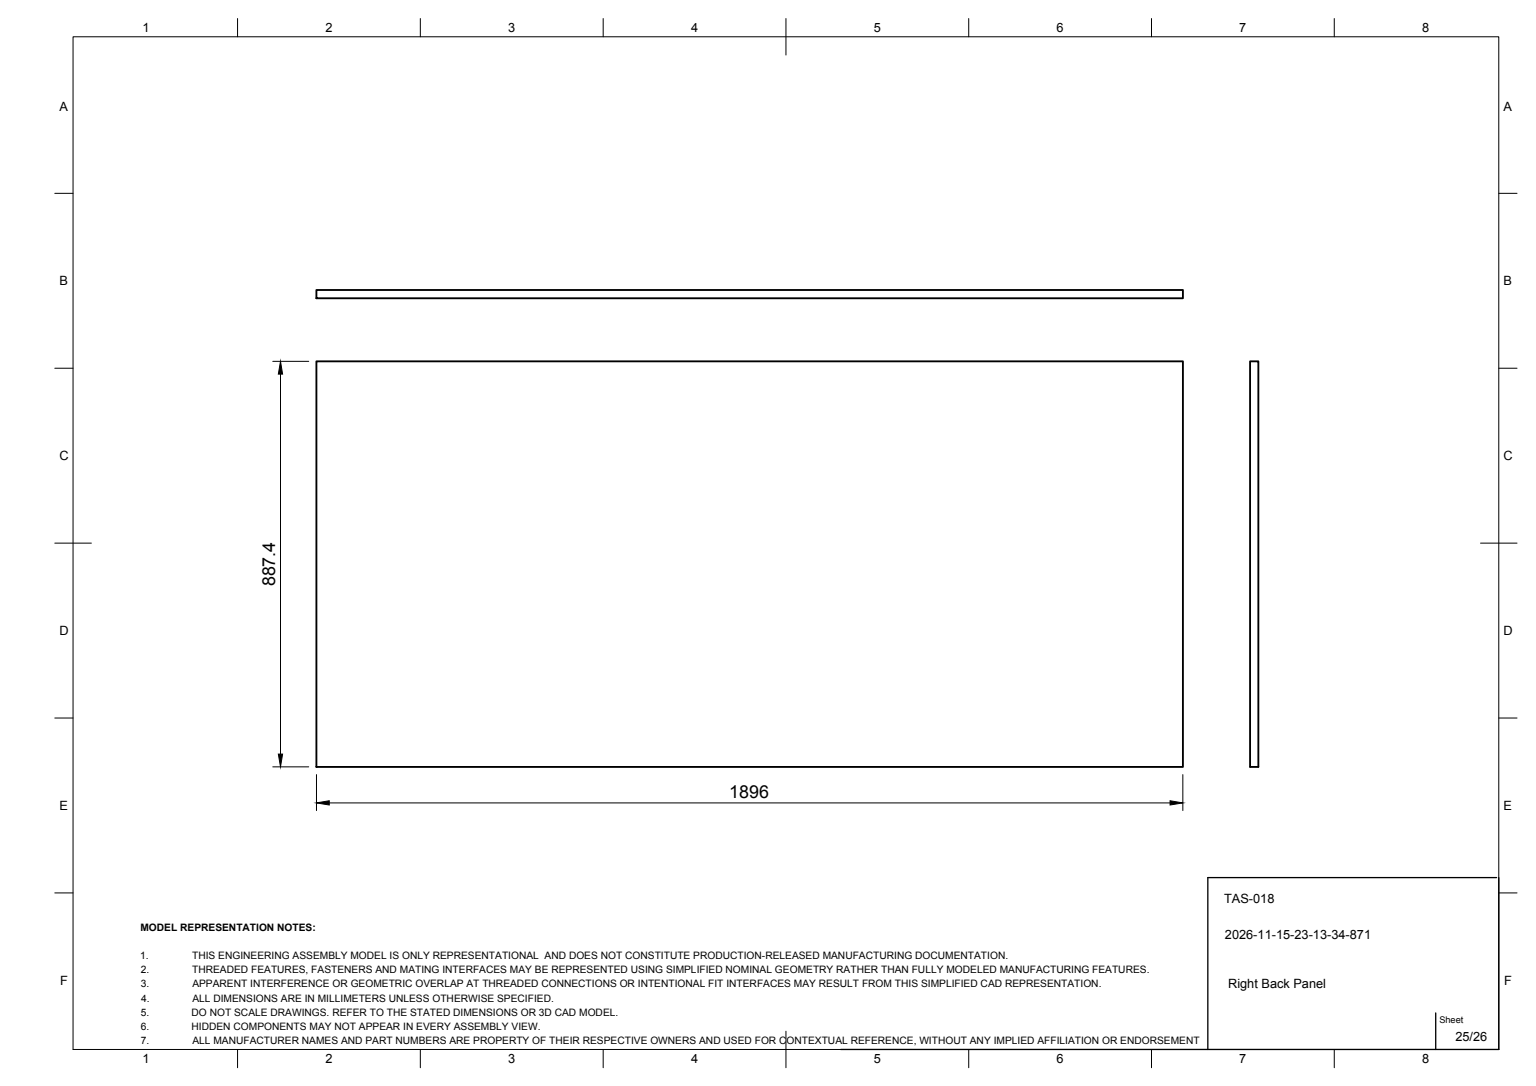
ISO-10303-21;
HEADER;
/* Generated by software containing ST-Developer
 * from STEP Tools, Inc. (www.steptools.com) 
 */

FILE_DESCRIPTION(
/* description */ (''),
/* implementation_level */ '2;1');

FILE_NAME(
/* name */ 'Right Back Panel.step',
/* time_stamp */ '2026-11-15T15:17:57-08:00',
/* author */ (''),
/* organization */ (''),
/* preprocessor_version */ 'ST-DEVELOPER v20.2',
/* originating_system */ 'Autodesk Translation Framework v15.17.0.0',
/* authorisation */ '');

FILE_SCHEMA (('AUTOMOTIVE_DESIGN { 1 0 10303 214 3 1 1 }'));
ENDSEC;

DATA;
#10=MECHANICAL_DESIGN_GEOMETRIC_PRESENTATION_REPRESENTATION('',(#200),#3723);
#152=SHAPE_REPRESENTATION_RELATIONSHIP('SRR','None',#3833,#176);
#176=ADVANCED_BREP_SHAPE_REPRESENTATION('',(#224),#3722);
#200=STYLED_ITEM('',(#3949),#224);
#224=MANIFOLD_SOLID_BREP('Body1',#2048);
#345=FACE_OUTER_BOUND('',#471,.T.);
#346=FACE_OUTER_BOUND('',#472,.T.);
#347=FACE_OUTER_BOUND('',#473,.T.);
#348=FACE_OUTER_BOUND('',#474,.T.);
#349=FACE_OUTER_BOUND('',#475,.T.);
#350=FACE_OUTER_BOUND('',#476,.T.);
#471=EDGE_LOOP('',(#1755,#1756,#1757,#1758));
#472=EDGE_LOOP('',(#1759,#1760,#1761,#1762));
#473=EDGE_LOOP('',(#1763,#1764,#1765,#1766));
#474=EDGE_LOOP('',(#1767,#1768,#1769,#1770));
#475=EDGE_LOOP('',(#1771,#1772,#1773,#1774));
#476=EDGE_LOOP('',(#1775,#1776,#1777,#1778));
#687=LINE('',#3623,#909);
#688=LINE('',#3625,#910);
#689=LINE('',#3627,#911);
#690=LINE('',#3628,#912);
#691=LINE('',#3631,#913);
#692=LINE('',#3633,#914);
#693=LINE('',#3634,#915);
#694=LINE('',#3637,#916);
#695=LINE('',#3639,#917);
#696=LINE('',#3640,#918);
#697=LINE('',#3642,#919);
#698=LINE('',#3643,#920);
#909=VECTOR('',#3033,74.6456692913386);
#910=VECTOR('',#3034,0.708661417322834);
#911=VECTOR('',#3035,74.6456692913386);
#912=VECTOR('',#3036,0.708661417322834);
#913=VECTOR('',#3039,34.9370078740157);
#914=VECTOR('',#3040,0.708661417322834);
#915=VECTOR('',#3041,34.9370078740157);
#916=VECTOR('',#3044,74.6456692913386);
#917=VECTOR('',#3045,0.708661417322834);
#918=VECTOR('',#3046,74.6456692913386);
#919=VECTOR('',#3049,34.9370078740157);
#920=VECTOR('',#3050,34.9370078740157);
#1069=VERTEX_POINT('',#3621);
#1070=VERTEX_POINT('',#3622);
#1071=VERTEX_POINT('',#3624);
#1072=VERTEX_POINT('',#3626);
#1073=VERTEX_POINT('',#3630);
#1074=VERTEX_POINT('',#3632);
#1075=VERTEX_POINT('',#3636);
#1076=VERTEX_POINT('',#3638);
#1299=EDGE_CURVE('',#1069,#1070,#687,.T.);
#1300=EDGE_CURVE('',#1071,#1070,#688,.T.);
#1301=EDGE_CURVE('',#1072,#1071,#689,.T.);
#1302=EDGE_CURVE('',#1072,#1069,#690,.T.);
#1303=EDGE_CURVE('',#1070,#1073,#691,.T.);
#1304=EDGE_CURVE('',#1074,#1073,#692,.T.);
#1305=EDGE_CURVE('',#1071,#1074,#693,.T.);
#1306=EDGE_CURVE('',#1073,#1075,#694,.T.);
#1307=EDGE_CURVE('',#1076,#1075,#695,.T.);
#1308=EDGE_CURVE('',#1074,#1076,#696,.T.);
#1309=EDGE_CURVE('',#1075,#1069,#697,.T.);
#1310=EDGE_CURVE('',#1076,#1072,#698,.T.);
#1755=ORIENTED_EDGE('',*,*,#1299,.T.);
#1756=ORIENTED_EDGE('',*,*,#1300,.F.);
#1757=ORIENTED_EDGE('',*,*,#1301,.F.);
#1758=ORIENTED_EDGE('',*,*,#1302,.T.);
#1759=ORIENTED_EDGE('',*,*,#1303,.T.);
#1760=ORIENTED_EDGE('',*,*,#1304,.F.);
#1761=ORIENTED_EDGE('',*,*,#1305,.F.);
#1762=ORIENTED_EDGE('',*,*,#1300,.T.);
#1763=ORIENTED_EDGE('',*,*,#1306,.T.);
#1764=ORIENTED_EDGE('',*,*,#1307,.F.);
#1765=ORIENTED_EDGE('',*,*,#1308,.F.);
#1766=ORIENTED_EDGE('',*,*,#1304,.T.);
#1767=ORIENTED_EDGE('',*,*,#1309,.T.);
#1768=ORIENTED_EDGE('',*,*,#1302,.F.);
#1769=ORIENTED_EDGE('',*,*,#1310,.F.);
#1770=ORIENTED_EDGE('',*,*,#1307,.T.);
#1771=ORIENTED_EDGE('',*,*,#1301,.T.);
#1772=ORIENTED_EDGE('',*,*,#1305,.T.);
#1773=ORIENTED_EDGE('',*,*,#1308,.T.);
#1774=ORIENTED_EDGE('',*,*,#1310,.T.);
#1775=ORIENTED_EDGE('',*,*,#1299,.F.);
#1776=ORIENTED_EDGE('',*,*,#1309,.F.);
#1777=ORIENTED_EDGE('',*,*,#1306,.F.);
#1778=ORIENTED_EDGE('',*,*,#1303,.F.);
#1893=PLANE('',#2473);
#1894=PLANE('',#2474);
#1895=PLANE('',#2475);
#1896=PLANE('',#2476);
#1897=PLANE('',#2477);
#1898=PLANE('',#2478);
#2019=ADVANCED_FACE('',(#345),#1893,.F.);
#2020=ADVANCED_FACE('',(#346),#1894,.F.);
#2021=ADVANCED_FACE('',(#347),#1895,.F.);
#2022=ADVANCED_FACE('',(#348),#1896,.F.);
#2023=ADVANCED_FACE('',(#349),#1897,.F.);
#2024=ADVANCED_FACE('',(#350),#1898,.T.);
#2048=CLOSED_SHELL('',(#2019,#2020,#2021,#2022,#2023,#2024));
#2472=AXIS2_PLACEMENT_3D('',#3619,#3029,#3030);
#2473=AXIS2_PLACEMENT_3D('',#3620,#3031,#3032);
#2474=AXIS2_PLACEMENT_3D('',#3629,#3037,#3038);
#2475=AXIS2_PLACEMENT_3D('',#3635,#3042,#3043);
#2476=AXIS2_PLACEMENT_3D('',#3641,#3047,#3048);
#2477=AXIS2_PLACEMENT_3D('',#3644,#3051,#3052);
#2478=AXIS2_PLACEMENT_3D('',#3645,#3053,#3054);
#3029=DIRECTION('axis',(0.,0.,1.));
#3030=DIRECTION('refdir',(1.,0.,0.));
#3031=DIRECTION('center_axis',(1.,0.,0.));
#3032=DIRECTION('ref_axis',(0.,0.,-1.));
#3033=DIRECTION('',(0.,-1.,0.));
#3034=DIRECTION('',(0.,0.,-1.));
#3035=DIRECTION('',(0.,-1.,0.));
#3036=DIRECTION('',(0.,0.,-1.));
#3037=DIRECTION('center_axis',(0.,1.,0.));
#3038=DIRECTION('ref_axis',(0.,0.,1.));
#3039=DIRECTION('',(1.,0.,0.));
#3040=DIRECTION('',(0.,0.,-1.));
#3041=DIRECTION('',(1.,0.,0.));
#3042=DIRECTION('center_axis',(-1.,0.,0.));
#3043=DIRECTION('ref_axis',(0.,0.,1.));
#3044=DIRECTION('',(0.,1.,0.));
#3045=DIRECTION('',(0.,0.,-1.));
#3046=DIRECTION('',(0.,1.,0.));
#3047=DIRECTION('center_axis',(0.,-1.,0.));
#3048=DIRECTION('ref_axis',(0.,0.,-1.));
#3049=DIRECTION('',(-1.,0.,0.));
#3050=DIRECTION('',(-1.,0.,0.));
#3051=DIRECTION('center_axis',(0.,0.,-1.));
#3052=DIRECTION('ref_axis',(-1.,0.,0.));
#3053=DIRECTION('center_axis',(0.,0.,-1.));
#3054=DIRECTION('ref_axis',(-1.,0.,0.));
#3619=CARTESIAN_POINT('',(0.,0.,0.));
#3620=CARTESIAN_POINT('Origin',(0.354330708661416,4.64566929133858,0.708661417322834));
#3621=CARTESIAN_POINT('',(0.354330708661416,79.2913385826772,0.));
#3622=CARTESIAN_POINT('',(0.354330708661416,4.64566929133858,0.));
#3623=CARTESIAN_POINT('',(0.354330708661416,79.2913385826772,0.));
#3624=CARTESIAN_POINT('',(0.354330708661416,4.64566929133858,0.708661417322834));
#3625=CARTESIAN_POINT('',(0.354330708661416,4.64566929133858,0.708661417322834));
#3626=CARTESIAN_POINT('',(0.354330708661416,79.2913385826772,0.708661417322834));
#3627=CARTESIAN_POINT('',(0.354330708661416,79.2913385826772,0.708661417322834));
#3628=CARTESIAN_POINT('',(0.354330708661416,79.2913385826772,0.708661417322834));
#3629=CARTESIAN_POINT('Origin',(0.354330708661416,4.64566929133858,0.708661417322834));
#3630=CARTESIAN_POINT('',(35.2913385826772,4.64566929133858,0.));
#3631=CARTESIAN_POINT('',(0.354330708661416,4.64566929133858,0.));
#3632=CARTESIAN_POINT('',(35.2913385826772,4.64566929133858,0.708661417322834));
#3633=CARTESIAN_POINT('',(35.2913385826772,4.64566929133858,0.708661417322834));
#3634=CARTESIAN_POINT('',(0.354330708661416,4.64566929133858,0.708661417322834));
#3635=CARTESIAN_POINT('Origin',(35.2913385826772,4.64566929133858,0.708661417322834));
#3636=CARTESIAN_POINT('',(35.2913385826772,79.2913385826772,0.));
#3637=CARTESIAN_POINT('',(35.2913385826772,4.64566929133858,0.));
#3638=CARTESIAN_POINT('',(35.2913385826772,79.2913385826772,0.708661417322834));
#3639=CARTESIAN_POINT('',(35.2913385826772,79.2913385826772,0.708661417322834));
#3640=CARTESIAN_POINT('',(35.2913385826772,4.64566929133858,0.708661417322834));
#3641=CARTESIAN_POINT('Origin',(0.354330708661416,79.2913385826772,0.708661417322834));
#3642=CARTESIAN_POINT('',(35.2913385826772,79.2913385826772,0.));
#3643=CARTESIAN_POINT('',(35.2913385826772,79.2913385826772,0.708661417322834));
#3644=CARTESIAN_POINT('Origin',(0.,0.,0.708661417322834));
#3645=CARTESIAN_POINT('Origin',(0.,0.,0.));
#3695=UNCERTAINTY_MEASURE_WITH_UNIT(LENGTH_MEASURE(0.000393700787401575),
#3725,'DISTANCE_ACCURACY_VALUE',
'Maximum model space distance between geometric entities at asserted c
onnectivities');
#3696=UNCERTAINTY_MEASURE_WITH_UNIT(LENGTH_MEASURE(0.000393700787401575),
#3725,'DISTANCE_ACCURACY_VALUE',
'Maximum model space distance between geometric entities at asserted c
onnectivities');
#3722=(
GEOMETRIC_REPRESENTATION_CONTEXT(3)
GLOBAL_UNCERTAINTY_ASSIGNED_CONTEXT((#3695))
GLOBAL_UNIT_ASSIGNED_CONTEXT((#3725,#3729,#3730))
REPRESENTATION_CONTEXT('','3D')
);
#3723=(
GEOMETRIC_REPRESENTATION_CONTEXT(3)
GLOBAL_UNCERTAINTY_ASSIGNED_CONTEXT((#3696))
GLOBAL_UNIT_ASSIGNED_CONTEXT((#3725,#3729,#3730))
REPRESENTATION_CONTEXT('','3D')
);
#3724=DIMENSIONAL_EXPONENTS(1.,0.,0.,0.,0.,0.,0.);
#3725=(
CONVERSION_BASED_UNIT('inch',#3728)
LENGTH_UNIT()
NAMED_UNIT(#3724)
);
#3726=(
LENGTH_UNIT()
NAMED_UNIT(*)
SI_UNIT(.MILLI.,.METRE.)
);
#3728=LENGTH_MEASURE_WITH_UNIT(LENGTH_MEASURE(25.4),#3726);
#3729=(
NAMED_UNIT(*)
PLANE_ANGLE_UNIT()
SI_UNIT($,.RADIAN.)
);
#3730=(
NAMED_UNIT(*)
SI_UNIT($,.STERADIAN.)
SOLID_ANGLE_UNIT()
);
#3756=SHAPE_DEFINITION_REPRESENTATION(#3783,#3833);
#3783=PRODUCT_DEFINITION_SHAPE('',$,#3860);
#3833=SHAPE_REPRESENTATION('',(#2472),#3722);
#3834=PRODUCT_DEFINITION_CONTEXT('part definition',#3914,'design');
#3860=PRODUCT_DEFINITION('2026-11-15-23-13-34-871','Right Back Panel',#3886,
#3834);
#3886=PRODUCT_DEFINITION_FORMATION('',$,#3941);
#3914=APPLICATION_CONTEXT(
'Core Data for Automotive Mechanical Design Process');
#3915=PRODUCT_CONTEXT('part definition',#3914,'mechanical');
#3941=PRODUCT('2026-11-15-23-13-34-871','Right Back Panel',$,(#3915));
#3949=PRESENTATION_STYLE_ASSIGNMENT((#3957));
#3957=SURFACE_STYLE_USAGE(.BOTH.,#3965);
#3965=SURFACE_SIDE_STYLE('',(#3973));
#3973=SURFACE_STYLE_FILL_AREA(#3981);
#3981=FILL_AREA_STYLE('Sky Blue',(#3989));
#3989=FILL_AREA_STYLE_COLOUR('Sky Blue',#3997);
#3997=COLOUR_RGB('Sky Blue',0.529411764705882,0.807843137254902,0.92156862745098);
ENDSEC;
END-ISO-10303-21;
